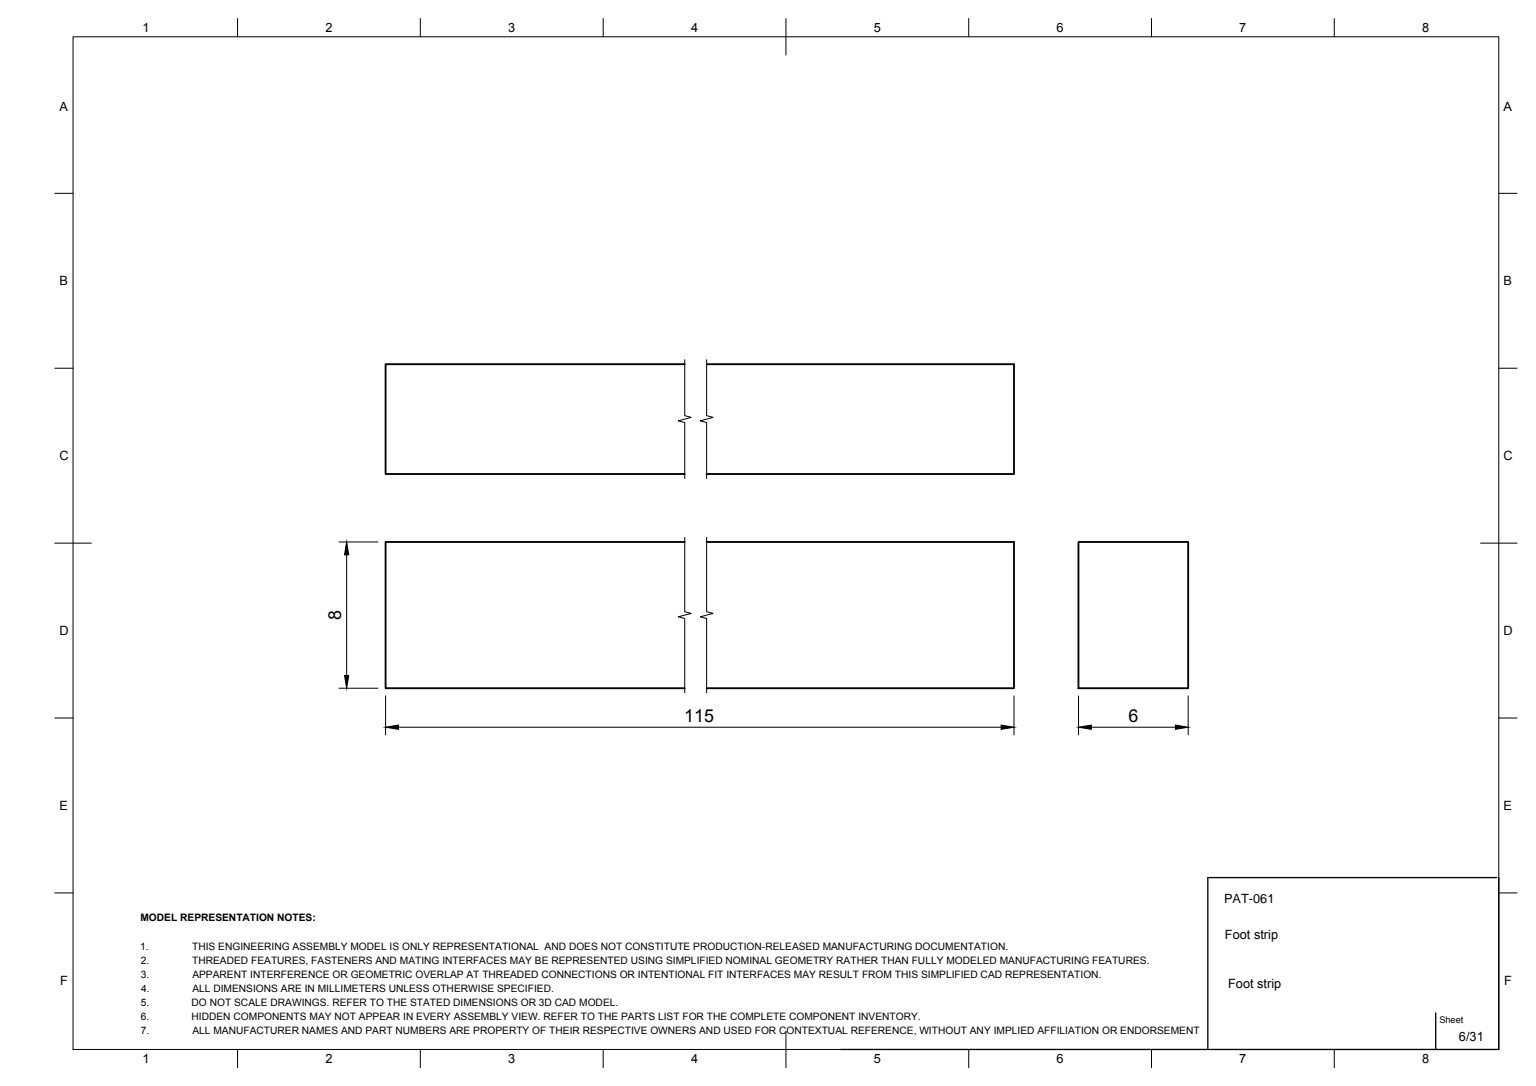
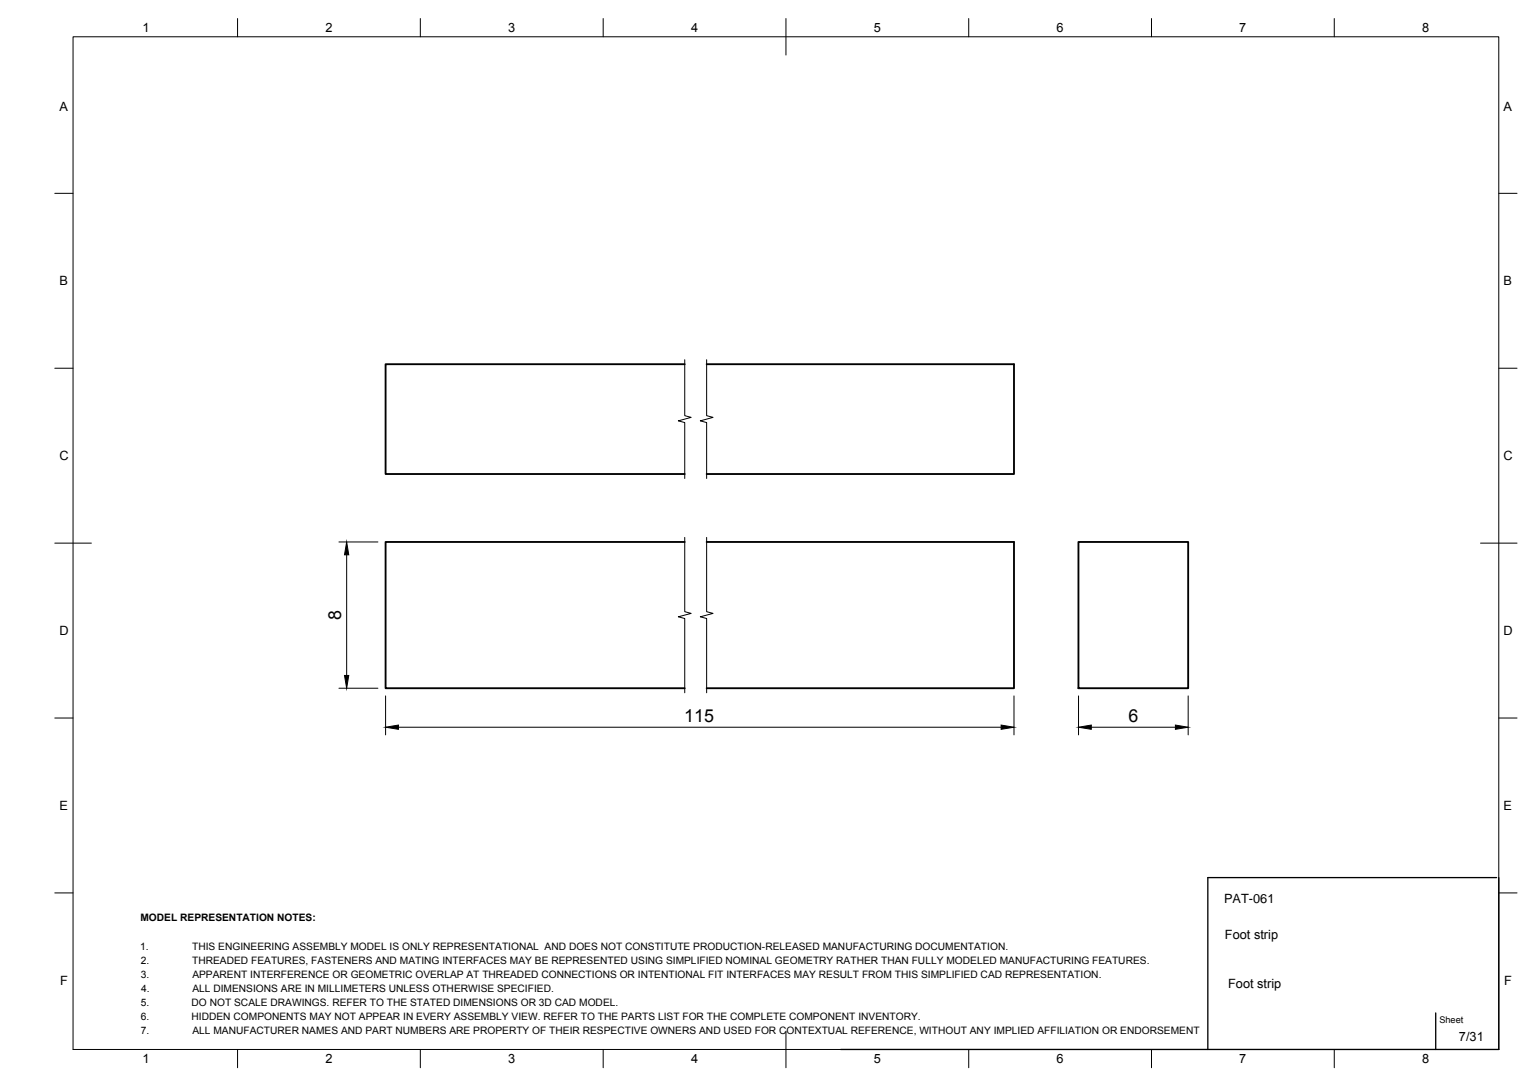
ISO-10303-21;
HEADER;
/* Generated by software containing ST-Developer
 * from STEP Tools, Inc. (www.steptools.com) 
 */

FILE_DESCRIPTION(
/* description */ ('Compact intermittent indexer'),
/* implementation_level */ '2;1');

FILE_NAME(
/* name */ 'Foot strip.step',
/* time_stamp */ '2026-10-29T16:32:17-07:00',
/* author */ (''),
/* organization */ (''),
/* preprocessor_version */ 'ST-DEVELOPER v20.2',
/* originating_system */ 'Autodesk Translation Framework v15.17.0.0',
/* authorisation */ '');

FILE_SCHEMA (('AUTOMOTIVE_DESIGN { 1 0 10303 214 3 1 1 }'));
ENDSEC;

DATA;
#10=MECHANICAL_DESIGN_GEOMETRIC_PRESENTATION_REPRESENTATION('',(#258),#10837);
#210=SHAPE_REPRESENTATION_RELATIONSHIP('SRR','None',#10944,#234);
#234=ADVANCED_BREP_SHAPE_REPRESENTATION('',(#290),#10811);
#258=STYLED_ITEM('',(#11152),#290);
#290=MANIFOLD_SOLID_BREP('Body1',#5630);
#502=PLANE('',#6051);
#503=PLANE('',#6052);
#504=PLANE('',#6053);
#505=PLANE('',#6054);
#506=PLANE('',#6055);
#507=PLANE('',#6056);
#713=FACE_OUTER_BOUND('',#1088,.T.);
#714=FACE_OUTER_BOUND('',#1089,.T.);
#715=FACE_OUTER_BOUND('',#1090,.T.);
#716=FACE_OUTER_BOUND('',#1091,.T.);
#717=FACE_OUTER_BOUND('',#1092,.T.);
#718=FACE_OUTER_BOUND('',#1093,.T.);
#1088=EDGE_LOOP('',(#3936,#3937,#3938,#3939));
#1089=EDGE_LOOP('',(#3940,#3941,#3942,#3943));
#1090=EDGE_LOOP('',(#3944,#3945,#3946,#3947));
#1091=EDGE_LOOP('',(#3948,#3949,#3950,#3951));
#1092=EDGE_LOOP('',(#3952,#3953,#3954,#3955));
#1093=EDGE_LOOP('',(#3956,#3957,#3958,#3959));
#1486=LINE('',#8824,#1844);
#1487=LINE('',#8826,#1845);
#1488=LINE('',#8828,#1846);
#1489=LINE('',#8829,#1847);
#1490=LINE('',#8832,#1848);
#1491=LINE('',#8834,#1849);
#1492=LINE('',#8835,#1850);
#1493=LINE('',#8838,#1851);
#1494=LINE('',#8840,#1852);
#1495=LINE('',#8841,#1853);
#1496=LINE('',#8843,#1854);
#1497=LINE('',#8844,#1855);
#1844=VECTOR('',#6968,1.);
#1845=VECTOR('',#6969,1.);
#1846=VECTOR('',#6970,1.);
#1847=VECTOR('',#6971,1.);
#1848=VECTOR('',#6974,1.);
#1849=VECTOR('',#6975,1.);
#1850=VECTOR('',#6976,1.);
#1851=VECTOR('',#6979,1.);
#1852=VECTOR('',#6980,1.);
#1853=VECTOR('',#6981,1.);
#1854=VECTOR('',#6984,1.);
#1855=VECTOR('',#6985,1.);
#2558=VERTEX_POINT('',#8822);
#2559=VERTEX_POINT('',#8823);
#2560=VERTEX_POINT('',#8825);
#2561=VERTEX_POINT('',#8827);
#2562=VERTEX_POINT('',#8831);
#2563=VERTEX_POINT('',#8833);
#2564=VERTEX_POINT('',#8837);
#2565=VERTEX_POINT('',#8839);
#3090=EDGE_CURVE('',#2558,#2559,#1486,.T.);
#3091=EDGE_CURVE('',#2559,#2560,#1487,.T.);
#3092=EDGE_CURVE('',#2561,#2560,#1488,.T.);
#3093=EDGE_CURVE('',#2558,#2561,#1489,.T.);
#3094=EDGE_CURVE('',#2562,#2558,#1490,.T.);
#3095=EDGE_CURVE('',#2563,#2561,#1491,.T.);
#3096=EDGE_CURVE('',#2562,#2563,#1492,.T.);
#3097=EDGE_CURVE('',#2564,#2562,#1493,.T.);
#3098=EDGE_CURVE('',#2565,#2563,#1494,.T.);
#3099=EDGE_CURVE('',#2564,#2565,#1495,.T.);
#3100=EDGE_CURVE('',#2559,#2564,#1496,.T.);
#3101=EDGE_CURVE('',#2560,#2565,#1497,.T.);
#3936=ORIENTED_EDGE('',*,*,#3090,.T.);
#3937=ORIENTED_EDGE('',*,*,#3091,.T.);
#3938=ORIENTED_EDGE('',*,*,#3092,.F.);
#3939=ORIENTED_EDGE('',*,*,#3093,.F.);
#3940=ORIENTED_EDGE('',*,*,#3094,.T.);
#3941=ORIENTED_EDGE('',*,*,#3093,.T.);
#3942=ORIENTED_EDGE('',*,*,#3095,.F.);
#3943=ORIENTED_EDGE('',*,*,#3096,.F.);
#3944=ORIENTED_EDGE('',*,*,#3097,.T.);
#3945=ORIENTED_EDGE('',*,*,#3096,.T.);
#3946=ORIENTED_EDGE('',*,*,#3098,.F.);
#3947=ORIENTED_EDGE('',*,*,#3099,.F.);
#3948=ORIENTED_EDGE('',*,*,#3100,.T.);
#3949=ORIENTED_EDGE('',*,*,#3099,.T.);
#3950=ORIENTED_EDGE('',*,*,#3101,.F.);
#3951=ORIENTED_EDGE('',*,*,#3091,.F.);
#3952=ORIENTED_EDGE('',*,*,#3101,.T.);
#3953=ORIENTED_EDGE('',*,*,#3098,.T.);
#3954=ORIENTED_EDGE('',*,*,#3095,.T.);
#3955=ORIENTED_EDGE('',*,*,#3092,.T.);
#3956=ORIENTED_EDGE('',*,*,#3100,.F.);
#3957=ORIENTED_EDGE('',*,*,#3090,.F.);
#3958=ORIENTED_EDGE('',*,*,#3094,.F.);
#3959=ORIENTED_EDGE('',*,*,#3097,.F.);
#5356=ADVANCED_FACE('',(#713),#502,.T.);
#5357=ADVANCED_FACE('',(#714),#503,.T.);
#5358=ADVANCED_FACE('',(#715),#504,.T.);
#5359=ADVANCED_FACE('',(#716),#505,.T.);
#5360=ADVANCED_FACE('',(#717),#506,.T.);
#5361=ADVANCED_FACE('',(#718),#507,.F.);
#5630=CLOSED_SHELL('',(#5356,#5357,#5358,#5359,#5360,#5361));
#6050=AXIS2_PLACEMENT_3D('',#8820,#6964,#6965);
#6051=AXIS2_PLACEMENT_3D('',#8821,#6966,#6967);
#6052=AXIS2_PLACEMENT_3D('',#8830,#6972,#6973);
#6053=AXIS2_PLACEMENT_3D('',#8836,#6977,#6978);
#6054=AXIS2_PLACEMENT_3D('',#8842,#6982,#6983);
#6055=AXIS2_PLACEMENT_3D('',#8845,#6986,#6987);
#6056=AXIS2_PLACEMENT_3D('',#8846,#6988,#6989);
#6964=DIRECTION('axis',(0.,0.,1.));
#6965=DIRECTION('refdir',(1.,0.,0.));
#6966=DIRECTION('center_axis',(0.,1.,0.));
#6967=DIRECTION('ref_axis',(-1.,0.,0.));
#6968=DIRECTION('',(-1.,0.,0.));
#6969=DIRECTION('',(0.,0.,1.));
#6970=DIRECTION('',(-1.,0.,0.));
#6971=DIRECTION('',(0.,0.,1.));
#6972=DIRECTION('center_axis',(1.,0.,0.));
#6973=DIRECTION('ref_axis',(0.,1.,0.));
#6974=DIRECTION('',(0.,1.,0.));
#6975=DIRECTION('',(0.,1.,0.));
#6976=DIRECTION('',(0.,0.,1.));
#6977=DIRECTION('center_axis',(0.,-1.,0.));
#6978=DIRECTION('ref_axis',(1.,0.,0.));
#6979=DIRECTION('',(1.,0.,0.));
#6980=DIRECTION('',(1.,0.,0.));
#6981=DIRECTION('',(0.,0.,1.));
#6982=DIRECTION('center_axis',(-1.,0.,0.));
#6983=DIRECTION('ref_axis',(0.,-1.,0.));
#6984=DIRECTION('',(0.,-1.,0.));
#6985=DIRECTION('',(0.,-1.,0.));
#6986=DIRECTION('center_axis',(0.,0.,1.));
#6987=DIRECTION('ref_axis',(1.,0.,0.));
#6988=DIRECTION('center_axis',(0.,0.,1.));
#6989=DIRECTION('ref_axis',(1.,0.,0.));
#8820=CARTESIAN_POINT('',(0.,0.,0.));
#8821=CARTESIAN_POINT('Origin',(8.,-3.2,-0.6));
#8822=CARTESIAN_POINT('',(8.,-3.2,-0.6));
#8823=CARTESIAN_POINT('',(-3.5,-3.2,-0.6));
#8824=CARTESIAN_POINT('',(8.,-3.2,-0.6));
#8825=CARTESIAN_POINT('',(-3.5,-3.2,0.));
#8826=CARTESIAN_POINT('',(-3.5,-3.2,-0.6));
#8827=CARTESIAN_POINT('',(8.,-3.2,0.));
#8828=CARTESIAN_POINT('',(8.,-3.2,0.));
#8829=CARTESIAN_POINT('',(8.,-3.2,-0.6));
#8830=CARTESIAN_POINT('Origin',(8.,-4.,-0.6));
#8831=CARTESIAN_POINT('',(8.,-4.,-0.6));
#8832=CARTESIAN_POINT('',(8.,-4.,-0.6));
#8833=CARTESIAN_POINT('',(8.,-4.,0.));
#8834=CARTESIAN_POINT('',(8.,-4.,0.));
#8835=CARTESIAN_POINT('',(8.,-4.,-0.6));
#8836=CARTESIAN_POINT('Origin',(-3.5,-4.,-0.6));
#8837=CARTESIAN_POINT('',(-3.5,-4.,-0.6));
#8838=CARTESIAN_POINT('',(-3.5,-4.,-0.6));
#8839=CARTESIAN_POINT('',(-3.5,-4.,0.));
#8840=CARTESIAN_POINT('',(-3.5,-4.,0.));
#8841=CARTESIAN_POINT('',(-3.5,-4.,-0.6));
#8842=CARTESIAN_POINT('Origin',(-3.5,-3.2,-0.6));
#8843=CARTESIAN_POINT('',(-3.5,-3.2,-0.6));
#8844=CARTESIAN_POINT('',(-3.5,-3.2,0.));
#8845=CARTESIAN_POINT('Origin',(2.25,-3.6,0.));
#8846=CARTESIAN_POINT('Origin',(2.25,-3.6,-0.6));
#10781=UNCERTAINTY_MEASURE_WITH_UNIT(LENGTH_MEASURE(0.001),#10838,
'DISTANCE_ACCURACY_VALUE',
'Maximum model space distance between geometric entities at asserted c
onnectivities');
#10807=UNCERTAINTY_MEASURE_WITH_UNIT(LENGTH_MEASURE(0.001),#10838,
'DISTANCE_ACCURACY_VALUE',
'Maximum model space distance between geometric entities at asserted c
onnectivities');
#10811=(
GEOMETRIC_REPRESENTATION_CONTEXT(3)
GLOBAL_UNCERTAINTY_ASSIGNED_CONTEXT((#10781))
GLOBAL_UNIT_ASSIGNED_CONTEXT((#10838,#10840,#10841))
REPRESENTATION_CONTEXT('','3D')
);
#10837=(
GEOMETRIC_REPRESENTATION_CONTEXT(3)
GLOBAL_UNCERTAINTY_ASSIGNED_CONTEXT((#10807))
GLOBAL_UNIT_ASSIGNED_CONTEXT((#10838,#10840,#10841))
REPRESENTATION_CONTEXT('','3D')
);
#10838=(
LENGTH_UNIT()
NAMED_UNIT(*)
SI_UNIT(.CENTI.,.METRE.)
);
#10840=(
NAMED_UNIT(*)
PLANE_ANGLE_UNIT()
SI_UNIT($,.RADIAN.)
);
#10841=(
NAMED_UNIT(*)
SI_UNIT($,.STERADIAN.)
SOLID_ANGLE_UNIT()
);
#10845=SHAPE_DEFINITION_REPRESENTATION(#10874,#10944);
#10874=PRODUCT_DEFINITION_SHAPE('',$,#10974);
#10944=SHAPE_REPRESENTATION('',(#6050),#10811);
#10970=PRODUCT_DEFINITION_CONTEXT('part definition',#11059,'design');
#10974=PRODUCT_DEFINITION('Foot strip','Foot strip',#11003,#10970);
#11003=PRODUCT_DEFINITION_FORMATION('',$,#11064);
#11059=APPLICATION_CONTEXT(
'Core Data for Automotive Mechanical Design Process');
#11060=PRODUCT_CONTEXT('part definition',#11059,'mechanical');
#11064=PRODUCT('Foot strip','Foot strip','Foot strip',(#11060));
#11146=COLOUR_RGB('Light Blue',0.38,0.62,0.78);
#11147=FILL_AREA_STYLE_COLOUR('',#11146);
#11148=FILL_AREA_STYLE('',(#11147));
#11149=SURFACE_STYLE_FILL_AREA(#11148);
#11150=SURFACE_SIDE_STYLE('',(#11149));
#11151=SURFACE_STYLE_USAGE(.BOTH.,#11150);
#11152=PRESENTATION_STYLE_ASSIGNMENT((#11151));
ENDSEC;
END-ISO-10303-21;
